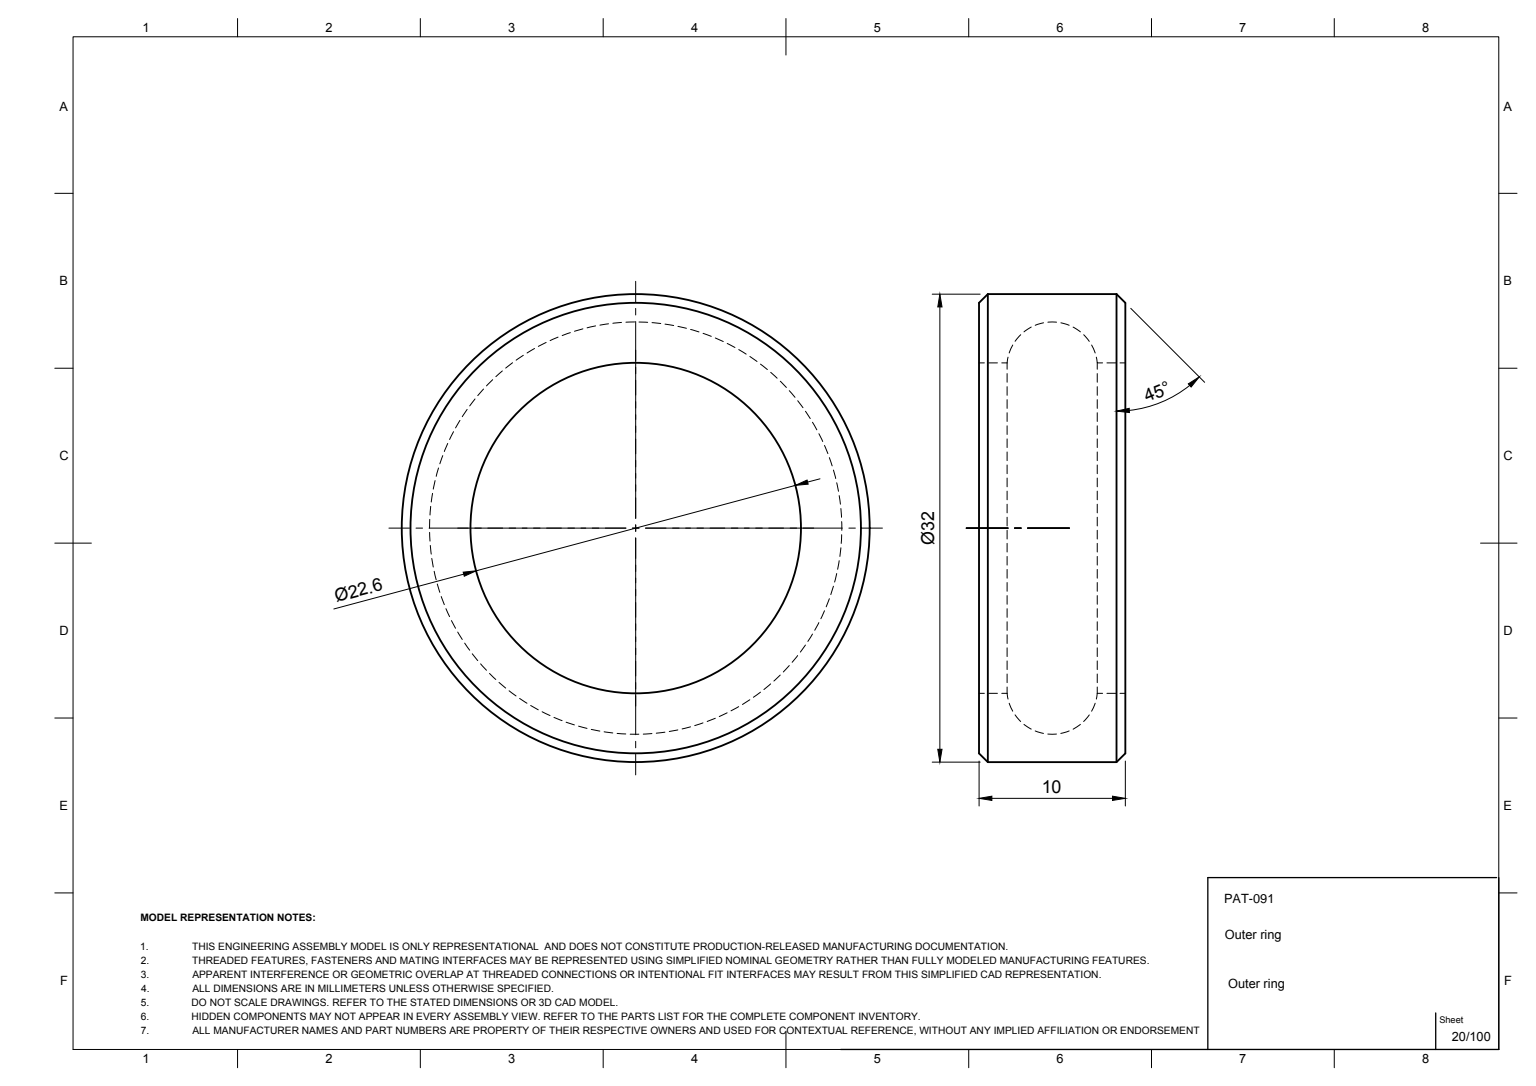
ISO-10303-21;
HEADER;
/* Generated by software containing ST-Developer
 * from STEP Tools, Inc. (www.steptools.com) 
 */

FILE_DESCRIPTION(
/* description */ ('PAT-091'),
/* implementation_level */ '2;1');

FILE_NAME(
/* name */ 'Outer ring.step',
/* time_stamp */ '2026-10-27T15:34:44-07:00',
/* author */ (''),
/* organization */ (''),
/* preprocessor_version */ 'ST-DEVELOPER v20.2',
/* originating_system */ 'Autodesk Translation Framework v15.17.0.0',
/* authorisation */ '');

FILE_SCHEMA (('AUTOMOTIVE_DESIGN { 1 0 10303 214 3 1 1 }'));
ENDSEC;

DATA;
#10=MECHANICAL_DESIGN_GEOMETRIC_PRESENTATION_REPRESENTATION('',(#1071),#25100);
#36=TOROIDAL_SURFACE('',#16154,1.1,0.309556);
#743=CONICAL_SURFACE('',#16165,1.57,0.785398163397449);
#744=CONICAL_SURFACE('',#16169,1.57,0.785398163397449);
#851=SHAPE_REPRESENTATION_RELATIONSHIP('SRR','None',#25619,#961);
#961=ADVANCED_BREP_SHAPE_REPRESENTATION('',(#1192),#25089);
#1071=STYLED_ITEM('',(#26191),#1192);
#1192=MANIFOLD_SOLID_BREP('Body1',#13351);
#1619=FACE_BOUND('',#4008,.T.);
#1620=FACE_BOUND('',#4013,.T.);
#2026=PLANE('',#16162);
#2027=PLANE('',#16171);
#2783=FACE_OUTER_BOUND('',#4005,.T.);
#2784=FACE_OUTER_BOUND('',#4006,.T.);
#2785=FACE_OUTER_BOUND('',#4007,.T.);
#2786=FACE_OUTER_BOUND('',#4009,.T.);
#2787=FACE_OUTER_BOUND('',#4010,.T.);
#2788=FACE_OUTER_BOUND('',#4011,.T.);
#2789=FACE_OUTER_BOUND('',#4012,.T.);
#2790=FACE_OUTER_BOUND('',#4014,.T.);
#4005=EDGE_LOOP('',(#11740,#11741,#11742,#11743,#11744,#11745));
#4006=EDGE_LOOP('',(#11746,#11747,#11748,#11749,#11750));
#4007=EDGE_LOOP('',(#11751));
#4008=EDGE_LOOP('',(#11752));
#4009=EDGE_LOOP('',(#11753,#11754,#11755,#11756));
#4010=EDGE_LOOP('',(#11757,#11758,#11759,#11760));
#4011=EDGE_LOOP('',(#11761,#11762,#11763,#11764));
#4012=EDGE_LOOP('',(#11765));
#4013=EDGE_LOOP('',(#11766));
#4014=EDGE_LOOP('',(#11767,#11768,#11769,#11770,#11771));
#4839=LINE('',#24245,#5579);
#4840=LINE('',#24254,#5580);
#4841=LINE('',#24258,#5581);
#4842=LINE('',#24262,#5582);
#4843=LINE('',#24265,#5583);
#5579=VECTOR('',#20337,1.129765);
#5580=VECTOR('',#20348,1.57);
#5581=VECTOR('',#20353,1.6);
#5582=VECTOR('',#20358,1.57);
#5583=VECTOR('',#20363,1.129765);
#6269=CIRCLE('',#16155,1.129765);
#6270=CIRCLE('',#16156,1.129765);
#6271=CIRCLE('',#16157,0.309556);
#6272=CIRCLE('',#16158,1.129765);
#6273=CIRCLE('',#16159,1.129765);
#6274=CIRCLE('',#16161,1.129765);
#6275=CIRCLE('',#16163,1.54);
#6276=CIRCLE('',#16164,1.129765);
#6277=CIRCLE('',#16166,1.6);
#6278=CIRCLE('',#16168,1.6);
#6279=CIRCLE('',#16170,1.54);
#7301=VERTEX_POINT('',#24233);
#7302=VERTEX_POINT('',#24234);
#7303=VERTEX_POINT('',#24237);
#7304=VERTEX_POINT('',#24239);
#7305=VERTEX_POINT('',#24243);
#7306=VERTEX_POINT('',#24247);
#7307=VERTEX_POINT('',#24249);
#7308=VERTEX_POINT('',#24252);
#7309=VERTEX_POINT('',#24256);
#7310=VERTEX_POINT('',#24260);
#8805=EDGE_CURVE('',#7301,#7302,#6269,.T.);
#8806=EDGE_CURVE('',#7302,#7301,#6270,.T.);
#8807=EDGE_CURVE('',#7302,#7303,#6271,.T.);
#8808=EDGE_CURVE('',#7304,#7303,#6272,.T.);
#8809=EDGE_CURVE('',#7303,#7304,#6273,.T.);
#8810=EDGE_CURVE('',#7305,#7305,#6274,.T.);
#8811=EDGE_CURVE('',#7305,#7304,#4839,.T.);
#8812=EDGE_CURVE('',#7306,#7306,#6275,.T.);
#8813=EDGE_CURVE('',#7307,#7307,#6276,.T.);
#8814=EDGE_CURVE('',#7308,#7308,#6277,.T.);
#8815=EDGE_CURVE('',#7308,#7306,#4840,.T.);
#8816=EDGE_CURVE('',#7309,#7309,#6278,.T.);
#8817=EDGE_CURVE('',#7309,#7308,#4841,.T.);
#8818=EDGE_CURVE('',#7310,#7310,#6279,.T.);
#8819=EDGE_CURVE('',#7310,#7309,#4842,.T.);
#8820=EDGE_CURVE('',#7301,#7307,#4843,.T.);
#11740=ORIENTED_EDGE('',*,*,#8805,.F.);
#11741=ORIENTED_EDGE('',*,*,#8806,.F.);
#11742=ORIENTED_EDGE('',*,*,#8807,.T.);
#11743=ORIENTED_EDGE('',*,*,#8808,.F.);
#11744=ORIENTED_EDGE('',*,*,#8809,.F.);
#11745=ORIENTED_EDGE('',*,*,#8807,.F.);
#11746=ORIENTED_EDGE('',*,*,#8810,.T.);
#11747=ORIENTED_EDGE('',*,*,#8811,.T.);
#11748=ORIENTED_EDGE('',*,*,#8808,.T.);
#11749=ORIENTED_EDGE('',*,*,#8809,.T.);
#11750=ORIENTED_EDGE('',*,*,#8811,.F.);
#11751=ORIENTED_EDGE('',*,*,#8812,.F.);
#11752=ORIENTED_EDGE('',*,*,#8813,.T.);
#11753=ORIENTED_EDGE('',*,*,#8814,.F.);
#11754=ORIENTED_EDGE('',*,*,#8815,.T.);
#11755=ORIENTED_EDGE('',*,*,#8812,.T.);
#11756=ORIENTED_EDGE('',*,*,#8815,.F.);
#11757=ORIENTED_EDGE('',*,*,#8816,.F.);
#11758=ORIENTED_EDGE('',*,*,#8817,.T.);
#11759=ORIENTED_EDGE('',*,*,#8814,.T.);
#11760=ORIENTED_EDGE('',*,*,#8817,.F.);
#11761=ORIENTED_EDGE('',*,*,#8818,.F.);
#11762=ORIENTED_EDGE('',*,*,#8819,.T.);
#11763=ORIENTED_EDGE('',*,*,#8816,.T.);
#11764=ORIENTED_EDGE('',*,*,#8819,.F.);
#11765=ORIENTED_EDGE('',*,*,#8818,.T.);
#11766=ORIENTED_EDGE('',*,*,#8810,.F.);
#11767=ORIENTED_EDGE('',*,*,#8805,.T.);
#11768=ORIENTED_EDGE('',*,*,#8806,.T.);
#11769=ORIENTED_EDGE('',*,*,#8820,.T.);
#11770=ORIENTED_EDGE('',*,*,#8813,.F.);
#11771=ORIENTED_EDGE('',*,*,#8820,.F.);
#12393=CYLINDRICAL_SURFACE('',#16160,1.129765);
#12394=CYLINDRICAL_SURFACE('',#16167,1.6);
#12395=CYLINDRICAL_SURFACE('',#16172,1.129765);
#13150=ADVANCED_FACE('',(#2783),#36,.F.);
#13151=ADVANCED_FACE('',(#2784),#12393,.F.);
#13152=ADVANCED_FACE('',(#2785,#1619),#2026,.T.);
#13153=ADVANCED_FACE('',(#2786),#743,.T.);
#13154=ADVANCED_FACE('',(#2787),#12394,.T.);
#13155=ADVANCED_FACE('',(#2788),#744,.T.);
#13156=ADVANCED_FACE('',(#2789,#1620),#2027,.T.);
#13157=ADVANCED_FACE('',(#2790),#12395,.F.);
#13351=CLOSED_SHELL('',(#13150,#13151,#13152,#13153,#13154,#13155,#13156,
#13157));
#16153=AXIS2_PLACEMENT_3D('',#24231,#20319,#20320);
#16154=AXIS2_PLACEMENT_3D('',#24232,#20321,#20322);
#16155=AXIS2_PLACEMENT_3D('',#24235,#20323,#20324);
#16156=AXIS2_PLACEMENT_3D('',#24236,#20325,#20326);
#16157=AXIS2_PLACEMENT_3D('',#24238,#20327,#20328);
#16158=AXIS2_PLACEMENT_3D('',#24240,#20329,#20330);
#16159=AXIS2_PLACEMENT_3D('',#24241,#20331,#20332);
#16160=AXIS2_PLACEMENT_3D('',#24242,#20333,#20334);
#16161=AXIS2_PLACEMENT_3D('',#24244,#20335,#20336);
#16162=AXIS2_PLACEMENT_3D('',#24246,#20338,#20339);
#16163=AXIS2_PLACEMENT_3D('',#24248,#20340,#20341);
#16164=AXIS2_PLACEMENT_3D('',#24250,#20342,#20343);
#16165=AXIS2_PLACEMENT_3D('',#24251,#20344,#20345);
#16166=AXIS2_PLACEMENT_3D('',#24253,#20346,#20347);
#16167=AXIS2_PLACEMENT_3D('',#24255,#20349,#20350);
#16168=AXIS2_PLACEMENT_3D('',#24257,#20351,#20352);
#16169=AXIS2_PLACEMENT_3D('',#24259,#20354,#20355);
#16170=AXIS2_PLACEMENT_3D('',#24261,#20356,#20357);
#16171=AXIS2_PLACEMENT_3D('',#24263,#20359,#20360);
#16172=AXIS2_PLACEMENT_3D('',#24264,#20361,#20362);
#20319=DIRECTION('axis',(0.,0.,1.));
#20320=DIRECTION('refdir',(1.,0.,0.));
#20321=DIRECTION('center_axis',(0.,-1.,0.));
#20322=DIRECTION('ref_axis',(0.,0.,-1.));
#20323=DIRECTION('center_axis',(0.,-1.,0.));
#20324=DIRECTION('ref_axis',(1.,0.,0.));
#20325=DIRECTION('center_axis',(0.,-1.,0.));
#20326=DIRECTION('ref_axis',(1.,0.,0.));
#20327=DIRECTION('center_axis',(1.,0.,1.22464679914735E-16));
#20328=DIRECTION('ref_axis',(-1.22464679914735E-16,0.,1.));
#20329=DIRECTION('center_axis',(0.,1.,0.));
#20330=DIRECTION('ref_axis',(1.,0.,0.));
#20331=DIRECTION('center_axis',(0.,1.,0.));
#20332=DIRECTION('ref_axis',(1.,0.,0.));
#20333=DIRECTION('center_axis',(0.,-1.,0.));
#20334=DIRECTION('ref_axis',(1.,0.,0.));
#20335=DIRECTION('center_axis',(0.,-1.,0.));
#20336=DIRECTION('ref_axis',(1.,0.,0.));
#20337=DIRECTION('',(0.,1.,0.));
#20338=DIRECTION('center_axis',(0.,1.,0.));
#20339=DIRECTION('ref_axis',(0.,0.,1.));
#20340=DIRECTION('center_axis',(0.,-1.,0.));
#20341=DIRECTION('ref_axis',(1.,0.,0.));
#20342=DIRECTION('center_axis',(0.,-1.,0.));
#20343=DIRECTION('ref_axis',(1.,0.,0.));
#20344=DIRECTION('center_axis',(0.,-1.,0.));
#20345=DIRECTION('ref_axis',(1.,0.,0.));
#20346=DIRECTION('center_axis',(0.,-1.,0.));
#20347=DIRECTION('ref_axis',(1.,0.,0.));
#20348=DIRECTION('',(0.707106781186548,0.707106781186547,8.65956056235494E-17));
#20349=DIRECTION('center_axis',(0.,-1.,0.));
#20350=DIRECTION('ref_axis',(1.,0.,0.));
#20351=DIRECTION('center_axis',(0.,-1.,0.));
#20352=DIRECTION('ref_axis',(1.,0.,0.));
#20353=DIRECTION('',(0.,1.,0.));
#20354=DIRECTION('center_axis',(0.,1.,0.));
#20355=DIRECTION('ref_axis',(1.,0.,0.));
#20356=DIRECTION('center_axis',(0.,-1.,0.));
#20357=DIRECTION('ref_axis',(1.,0.,0.));
#20358=DIRECTION('',(-0.707106781186548,0.707106781186547,-8.65956056235494E-17));
#20359=DIRECTION('center_axis',(0.,-1.,0.));
#20360=DIRECTION('ref_axis',(0.,0.,-1.));
#20361=DIRECTION('center_axis',(0.,-1.,0.));
#20362=DIRECTION('ref_axis',(1.,0.,0.));
#20363=DIRECTION('',(0.,1.,0.));
#24231=CARTESIAN_POINT('',(0.,0.,0.));
#24232=CARTESIAN_POINT('Origin',(0.,0.,0.));
#24233=CARTESIAN_POINT('',(-1.129765,0.308121667383195,-1.38356309103871E-16));
#24234=CARTESIAN_POINT('',(-1.38356309103871E-16,0.308121667383195,1.129765));
#24235=CARTESIAN_POINT('Origin',(0.,0.308121667383195,0.));
#24236=CARTESIAN_POINT('Origin',(0.,0.308121667383195,0.));
#24237=CARTESIAN_POINT('',(-1.38356309103871E-16,-0.308121667383195,1.129765));
#24238=CARTESIAN_POINT('Origin',(-1.34711147906209E-16,0.,1.1));
#24239=CARTESIAN_POINT('',(-1.129765,-0.308121667383195,1.38356309103871E-16));
#24240=CARTESIAN_POINT('Origin',(0.,-0.308121667383195,0.));
#24241=CARTESIAN_POINT('Origin',(0.,-0.308121667383195,0.));
#24242=CARTESIAN_POINT('Origin',(0.,0.,0.));
#24243=CARTESIAN_POINT('',(-1.129765,-0.5,-1.38356309103871E-16));
#24244=CARTESIAN_POINT('Origin',(0.,-0.5,0.));
#24245=CARTESIAN_POINT('',(-1.129765,0.,-1.38356309103871E-16));
#24246=CARTESIAN_POINT('Origin',(1.54,0.5,0.));
#24247=CARTESIAN_POINT('',(-1.54,0.5,-1.88595607068692E-16));
#24248=CARTESIAN_POINT('Origin',(0.,0.5,0.));
#24249=CARTESIAN_POINT('',(-1.129765,0.5,-1.38356309103871E-16));
#24250=CARTESIAN_POINT('Origin',(0.,0.5,0.));
#24251=CARTESIAN_POINT('Origin',(0.,0.47,0.));
#24252=CARTESIAN_POINT('',(-1.6,0.44,-1.95943487863577E-16));
#24253=CARTESIAN_POINT('Origin',(0.,0.44,0.));
#24254=CARTESIAN_POINT('',(-1.57,0.47,-1.92269547466134E-16));
#24255=CARTESIAN_POINT('Origin',(0.,0.,0.));
#24256=CARTESIAN_POINT('',(-1.6,-0.44,-1.95943487863577E-16));
#24257=CARTESIAN_POINT('Origin',(0.,-0.44,0.));
#24258=CARTESIAN_POINT('',(-1.6,0.,-1.95943487863577E-16));
#24259=CARTESIAN_POINT('Origin',(0.,-0.47,0.));
#24260=CARTESIAN_POINT('',(-1.54,-0.5,-1.88595607068692E-16));
#24261=CARTESIAN_POINT('Origin',(0.,-0.5,0.));
#24262=CARTESIAN_POINT('',(-1.57,-0.47,-1.92269547466134E-16));
#24263=CARTESIAN_POINT('Origin',(1.129765,-0.5,0.));
#24264=CARTESIAN_POINT('Origin',(0.,0.,0.));
#24265=CARTESIAN_POINT('',(-1.129765,0.,-1.38356309103871E-16));
#24968=UNCERTAINTY_MEASURE_WITH_UNIT(LENGTH_MEASURE(0.001),#25101,
'DISTANCE_ACCURACY_VALUE',
'Maximum model space distance between geometric entities at asserted c
onnectivities');
#24979=UNCERTAINTY_MEASURE_WITH_UNIT(LENGTH_MEASURE(0.001),#25101,
'DISTANCE_ACCURACY_VALUE',
'Maximum model space distance between geometric entities at asserted c
onnectivities');
#25089=(
GEOMETRIC_REPRESENTATION_CONTEXT(3)
GLOBAL_UNCERTAINTY_ASSIGNED_CONTEXT((#24968))
GLOBAL_UNIT_ASSIGNED_CONTEXT((#25101,#25103,#25104))
REPRESENTATION_CONTEXT('','3D')
);
#25100=(
GEOMETRIC_REPRESENTATION_CONTEXT(3)
GLOBAL_UNCERTAINTY_ASSIGNED_CONTEXT((#24979))
GLOBAL_UNIT_ASSIGNED_CONTEXT((#25101,#25103,#25104))
REPRESENTATION_CONTEXT('','3D')
);
#25101=(
LENGTH_UNIT()
NAMED_UNIT(*)
SI_UNIT(.CENTI.,.METRE.)
);
#25103=(
NAMED_UNIT(*)
PLANE_ANGLE_UNIT()
SI_UNIT($,.RADIAN.)
);
#25104=(
NAMED_UNIT(*)
SI_UNIT($,.STERADIAN.)
SOLID_ANGLE_UNIT()
);
#25214=SHAPE_DEFINITION_REPRESENTATION(#25408,#25619);
#25408=PRODUCT_DEFINITION_SHAPE('',$,#25740);
#25619=SHAPE_REPRESENTATION('',(#16153),#25089);
#25630=PRODUCT_DEFINITION_CONTEXT('part definition',#25992,'design');
#25740=PRODUCT_DEFINITION('Outer ring','Outer ring',#25860,#25630);
#25860=PRODUCT_DEFINITION_FORMATION('',$,#26103);
#25992=APPLICATION_CONTEXT(
'Core Data for Automotive Mechanical Design Process');
#25993=PRODUCT_CONTEXT('part definition',#25992,'mechanical');
#26103=PRODUCT('Outer ring','Outer ring','Outer ring',(#25993));
#26185=COLOUR_RGB('Grey',0.48,0.52,0.57);
#26186=FILL_AREA_STYLE_COLOUR('',#26185);
#26187=FILL_AREA_STYLE('',(#26186));
#26188=SURFACE_STYLE_FILL_AREA(#26187);
#26189=SURFACE_SIDE_STYLE('',(#26188));
#26190=SURFACE_STYLE_USAGE(.BOTH.,#26189);
#26191=PRESENTATION_STYLE_ASSIGNMENT((#26190));
ENDSEC;
END-ISO-10303-21;
